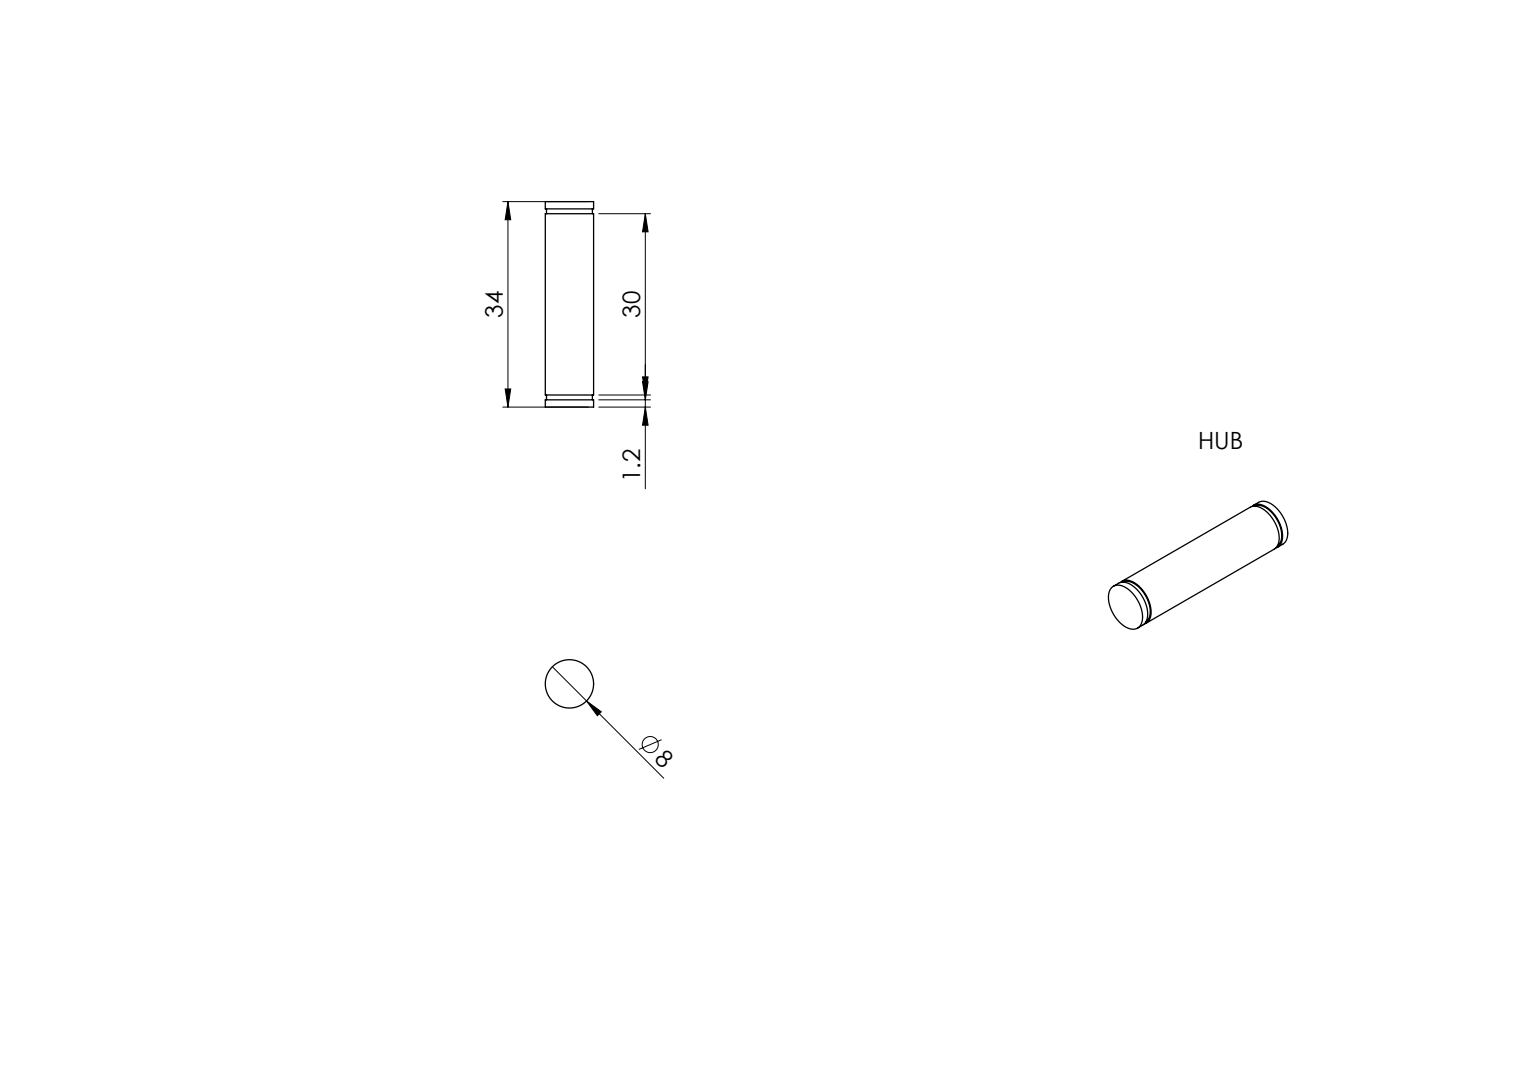
ISO-10303-21;
HEADER;
FILE_DESCRIPTION (('STEP AP214'),
    '1' );
FILE_NAME ('hub.step',
    '2026-10-31T03:44:21',
    ( '' ),
    ( '' ),
    'SwSTEP 2.0',
    'SolidWorks 2026',
    '' );
FILE_SCHEMA (( 'AUTOMOTIVE_DESIGN' ));
ENDSEC;

DATA;
#3=DIRECTION ( 'NONE',  ( -0.9999670257950099561, -0.008120795692649453515, 0.000000000000000000 ) ) ;
#38=VECTOR ( 'NONE', #9468, 1000.000000000000000 ) ;
#87=CARTESIAN_POINT ( 'NONE',  ( -155.0676494111543491, -18.79939778875158396, -15.79999999999999893 ) ) ;
#88=VERTEX_POINT ( 'NONE', #4235 ) ;
#158=AXIS2_PLACEMENT_3D ( 'NONE', #16967, #16677, #18346 ) ;
#163=DIRECTION ( 'NONE',  ( -0.9999670257950099561, -0.008120795692649453515, 0.000000000000000000 ) ) ;
#175=DIRECTION ( 'NONE',  ( 1.000000000000000000, 0.000000000000000000, 0.000000000000000000 ) ) ;
#223=DIRECTION ( 'NONE',  ( 2.191393683118470056E-17, 7.538405132783724027E-17, 1.000000000000000000 ) ) ;
#238=AXIS2_PLACEMENT_3D ( 'NONE', #6880, #15913, #19069 ) ;
#251=CIRCLE ( 'NONE', #8059, 3.800000000000000266 ) ;
#262=CARTESIAN_POINT ( 'NONE',  ( -154.9999999999999716, -14.99999999999999645, 15.79999999999999893 ) ) ;
#295=EDGE_CURVE ( 'NONE', #1806, #3807, #8927, .T. ) ;
#353=AXIS2_PLACEMENT_3D ( 'NONE', #12946, #2182, #2381 ) ;
#385=FACE_OUTER_BOUND ( 'NONE', #2616, .T. ) ;
#398=DIRECTION ( 'NONE',  ( 0.000000000000000000, 0.000000000000000000, 1.000000000000000000 ) ) ;
#423=EDGE_CURVE ( 'NONE', #3823, #976, #17703, .T. ) ;
#435=VECTOR ( 'NONE', #5633, 1000.000000000000000 ) ;
#465=EDGE_CURVE ( 'NONE', #17166, #14477, #13781, .T. ) ;
#471=ORIENTED_EDGE ( 'NONE', *, *, #4498, .F. ) ;
#479=DIRECTION ( 'NONE',  ( 0.9999419836444144449, 0.01077169184824096695, 0.000000000000000000 ) ) ;
#516=AXIS2_PLACEMENT_3D ( 'NONE', #18287, #3472, #2000 ) ;
#573=DIRECTION ( 'NONE',  ( -0.02045300604585054485, -0.9997908153927441699, -2.853726094247054863E-17 ) ) ;
#577=DIRECTION ( 'NONE',  ( -0.9999670257950099561, -0.008120795692649453515, 0.000000000000000000 ) ) ;
#594=DIRECTION ( 'NONE',  ( -0.000000000000000000, -0.000000000000000000, -1.000000000000000000 ) ) ;
#670=EDGE_CURVE ( 'NONE', #10950, #14856, #10929, .T. ) ;
#719=( NAMED_UNIT ( * ) SI_UNIT ( $, .STERADIAN. ) SOLID_ANGLE_UNIT ( ) );
#771=AXIS2_PLACEMENT_3D ( 'NONE', #7468, #11769, #12166 ) ;
#778=DIRECTION ( 'NONE',  ( 0.9999419836444144449, 0.01077169184824096695, 0.000000000000000000 ) ) ;
#833=ORIENTED_EDGE ( 'NONE', *, *, #15508, .T. ) ;
#856=CARTESIAN_POINT ( 'NONE',  ( -154.8505191518487152, -18.79705879280739467, -15.00000000000000000 ) ) ;
#867=CIRCLE ( 'NONE', #238, 4.000000000000021316 ) ;
#876=ADVANCED_FACE ( 'NONE', ( #9941 ), #2806, .F. ) ;
#964=VECTOR ( 'NONE', #1344, 1000.000000000000000 ) ;
#976=VERTEX_POINT ( 'NONE', #18201 ) ;
#979=AXIS2_PLACEMENT_3D ( 'NONE', #2910, #7500, #10431 ) ;
#994=VECTOR ( 'NONE', #12505, 999.9999999999998863 ) ;
#1010=EDGE_CURVE ( 'NONE', #13080, #4857, #251, .T. ) ;
#1011=EDGE_CURVE ( 'NONE', #88, #15786, #6202, .T. ) ;
#1029=VERTEX_POINT ( 'NONE', #10903 ) ;
#1037=CARTESIAN_POINT ( 'NONE',  ( -154.9999999999999716, -14.99999999999999645, 15.79999999999999893 ) ) ;
#1163=DIRECTION ( 'NONE',  ( 0.9999419836444144449, 0.01077169184824073971, -2.272467923560868285E-17 ) ) ;
#1171=CARTESIAN_POINT ( 'NONE',  ( -159.0000000000000000, -14.99999999999999645, -15.00000000000000000 ) ) ;
#1237=ORIENTED_EDGE ( 'NONE', *, *, #13531, .F. ) ;
#1253=ORIENTED_EDGE ( 'NONE', *, *, #5246, .T. ) ;
#1277=CARTESIAN_POINT ( 'NONE',  ( -155.0712099064782876, -18.99936609342274707, -15.79999999999999538 ) ) ;
#1342=DIRECTION ( 'NONE',  ( 0.000000000000000000, -1.000000000000000000, 0.000000000000000000 ) ) ;
#1344=DIRECTION ( 'NONE',  ( 2.191393683118470056E-17, 7.538405132783724027E-17, 1.000000000000000000 ) ) ;
#1377=EDGE_CURVE ( 'NONE', #14477, #19163, #867, .T. ) ;
#1399=DIRECTION ( 'NONE',  ( 0.000000000000000000, -1.000000000000000000, 0.000000000000000000 ) ) ;
#1407=VECTOR ( 'NONE', #12245, 1000.000000000000000 ) ;
#1410=DIRECTION ( 'NONE',  ( -0.000000000000000000, -0.000000000000000000, -1.000000000000000000 ) ) ;
#1437=LINE ( 'NONE', #5948, #15809 ) ;
#1480=ADVANCED_BREP_SHAPE_REPRESENTATION ( '', ( #8823, #10359 ), #8423 ) ;
#1486=EDGE_CURVE ( 'NONE', #976, #17995, #14820, .T. ) ;
#1506=FILL_AREA_STYLE_COLOUR ( '', #10923 ) ;
#1520=CIRCLE ( 'NONE', #16559, 4.000000000000031086 ) ;
#1522=DIRECTION ( 'NONE',  ( 0.000000000000000000, -1.000000000000000000, 0.000000000000000000 ) ) ;
#1534=DIRECTION ( 'NONE',  ( -0.000000000000000000, -0.000000000000000000, -1.000000000000000000 ) ) ;
#1551=CIRCLE ( 'NONE', #9363, 3.800000000000000266 ) ;
#1571=EDGE_LOOP ( 'NONE', ( #18455, #8024, #11206, #15769 ) ) ;
#1699=CARTESIAN_POINT ( 'NONE',  ( -150.9999999999999432, -14.99999999999999645, -15.79999999999999538 ) ) ;
#1740=( GEOMETRIC_REPRESENTATION_CONTEXT ( 3 ) GLOBAL_UNCERTAINTY_ASSIGNED_CONTEXT ( ( #16964 ) ) GLOBAL_UNIT_ASSIGNED_CONTEXT ( ( #13852, #6690, #719 ) ) REPRESENTATION_CONTEXT ( 'NONE', 'WORKASPACE' ) );
#1747=LINE ( 'NONE', #17038, #38 ) ;
#1750=VERTEX_POINT ( 'NONE', #7058 ) ;
#1787=AXIS2_PLACEMENT_3D ( 'NONE', #1037, #18895, #5430 ) ;
#1806=VERTEX_POINT ( 'NONE', #8533 ) ;
#1827=AXIS2_PLACEMENT_3D ( 'NONE', #10171, #6070, #13414 ) ;
#1886=CARTESIAN_POINT ( 'NONE',  ( -150.9999999999999432, -14.99999999999999645, 17.00000000000000000 ) ) ;
#1932=AXIS2_PLACEMENT_3D ( 'NONE', #7610, #4581, #163 ) ;
#1993=ORIENTED_EDGE ( 'NONE', *, *, #14194, .F. ) ;
#2000=DIRECTION ( 'NONE',  ( 0.000000000000000000, -1.000000000000000000, 0.000000000000000000 ) ) ;
#2045=CARTESIAN_POINT ( 'NONE',  ( -154.8605857259444463, -18.79744172571344762, 15.79999999999999893 ) ) ;
#2053=CARTESIAN_POINT ( 'NONE',  ( -155.0777214229742071, -18.79920509849242549, 15.79999999999999893 ) ) ;
#2182=DIRECTION ( 'NONE',  ( -0.000000000000000000, -0.000000000000000000, -1.000000000000000000 ) ) ;
#2216=CARTESIAN_POINT ( 'NONE',  ( -151.2002204621512078, -14.95906757097668027, -15.79999999999999893 ) ) ;
#2253=DIRECTION ( 'NONE',  ( 2.191393683118470056E-17, 7.538405132783724027E-17, 1.000000000000000000 ) ) ;
#2273=ORIENTED_EDGE ( 'NONE', *, *, #14413, .F. ) ;
#2381=DIRECTION ( 'NONE',  ( -1.000000000000000000, 0.000000000000000000, 0.000000000000000000 ) ) ;
#2384=EDGE_CURVE ( 'NONE', #4462, #5527, #16668, .T. ) ;
#2404=EDGE_CURVE ( 'NONE', #17995, #15708, #18515, .T. ) ;
#2411=CARTESIAN_POINT ( 'NONE',  ( -154.8426517387881347, -18.99690399242885874, -15.79999999999999538 ) ) ;
#2415=ORIENTED_EDGE ( 'NONE', *, *, #3275, .T. ) ;
#2432=DIRECTION ( 'NONE',  ( -0.9999670257950099561, -0.008120795692649453515, 0.000000000000000000 ) ) ;
#2462=DIRECTION ( 'NONE',  ( -2.191393683118470056E-17, -7.538405132783724027E-17, -1.000000000000000000 ) ) ;
#2558=CARTESIAN_POINT ( 'NONE',  ( -154.9999999999999716, -14.99999999999999645, -15.00000000000000000 ) ) ;
#2600=CARTESIAN_POINT ( 'NONE',  ( -158.7997795378487353, -15.04093242902330907, -15.79999999999999893 ) ) ;
#2616=EDGE_LOOP ( 'NONE', ( #12882, #6834, #7414, #8836 ) ) ;
#2634=ORIENTED_EDGE ( 'NONE', *, *, #11770, .F. ) ;
#2662=DIRECTION ( 'NONE',  ( -0.03668796685672145313, 0.9993267699245927949, 2.695122805014889898E-17 ) ) ;
#2731=LINE ( 'NONE', #2918, #7805 ) ;
#2736=ORIENTED_EDGE ( 'NONE', *, *, #4601, .T. ) ;
#2746=DIRECTION ( 'NONE',  ( 0.000000000000000000, 0.000000000000000000, -1.000000000000000000 ) ) ;
#2758=ORIENTED_EDGE ( 'NONE', *, *, #1011, .F. ) ;
#2760=CARTESIAN_POINT ( 'NONE',  ( -154.8532481325730998, -18.99730707969839116, 15.79999999999999893 ) ) ;
#2774=EDGE_LOOP ( 'NONE', ( #1993, #2634, #2415, #14369 ) ) ;
#2781=CARTESIAN_POINT ( 'NONE',  ( -154.9999999999999716, -14.99999999999999645, -15.79999999999999538 ) ) ;
#2806=PLANE ( 'NONE',  #12919 ) ;
#2868=CARTESIAN_POINT ( 'NONE',  ( -150.9999999999999432, -14.99999999999999645, 15.00000000000000000 ) ) ;
#2870=CARTESIAN_POINT ( 'NONE',  ( -151.2001253019789431, -14.96914097636792818, 15.00000000000000000 ) ) ;
#2871=CARTESIAN_POINT ( 'NONE',  ( 0.000000000000000000, 0.000000000000000000, 0.000000000000000000 ) ) ;
#2888=APPLICATION_CONTEXT ( 'automotive_design' ) ;
#2910=CARTESIAN_POINT ( 'NONE',  ( -154.9999999999999716, -14.99999999999999645, 15.79999999999999893 ) ) ;
#2911=FACE_OUTER_BOUND ( 'NONE', #4695, .T. ) ;
#2918=CARTESIAN_POINT ( 'NONE',  ( -154.8605857259444463, -18.79744172571344762, 15.00000000000000000 ) ) ;
#2983=SURFACE_STYLE_USAGE ( .BOTH. , #10055 ) ;
#2986=MECHANICAL_DESIGN_GEOMETRIC_PRESENTATION_REPRESENTATION('',(#8613),#1740);
#3058=VECTOR ( 'NONE', #18196, 1000.000000000000000 ) ;
#3081=EDGE_CURVE ( 'NONE', #3823, #4857, #6620, .T. ) ;
#3086=FILL_AREA_STYLE ('',( #1506 ) ) ;
#3190=CARTESIAN_POINT ( 'NONE',  ( -154.8505191518487152, -18.79705879280739467, -15.79999999999999893 ) ) ;
#3220=CARTESIAN_POINT ( 'NONE',  ( -154.8505191518487152, -18.79705879280739467, -15.79999999999999893 ) ) ;
#3244=EDGE_CURVE ( 'NONE', #16758, #5231, #4518, .T. ) ;
#3275=EDGE_CURVE ( 'NONE', #3719, #8297, #11699, .T. ) ;
#3295=AXIS2_PLACEMENT_3D ( 'NONE', #16109, #6193, #5104 ) ;
#3303=ORIENTED_EDGE ( 'NONE', *, *, #295, .T. ) ;
#3313=CARTESIAN_POINT ( 'NONE',  ( -155.0777214229742071, -18.79920509849242549, 15.00000000000000000 ) ) ;
#3436=ORIENTED_EDGE ( 'NONE', *, *, #423, .F. ) ;
#3438=DIRECTION ( 'NONE',  ( 1.000000000000000000, 0.000000000000000000, 0.000000000000000000 ) ) ;
#3472=DIRECTION ( 'NONE',  ( 2.191393683118470056E-17, 7.538405132783724027E-17, 1.000000000000000000 ) ) ;
#3521=PLANE ( 'NONE',  #3915 ) ;
#3588=AXIS2_PLACEMENT_3D ( 'NONE', #2781, #4732, #1399 ) ;
#3592=CARTESIAN_POINT ( 'NONE',  ( -159.0000000000000000, -14.99999999999999645, 17.00000000000000000 ) ) ;
#3686=CARTESIAN_POINT ( 'NONE',  ( -154.8505191518487152, -18.79705879280739467, -15.79999999999999893 ) ) ;
#3719=VERTEX_POINT ( 'NONE', #8643 ) ;
#3744=ORIENTED_EDGE ( 'NONE', *, *, #6811, .F. ) ;
#3750=EDGE_CURVE ( 'NONE', #976, #4855, #11582, .T. ) ;
#3807=VERTEX_POINT ( 'NONE', #2600 ) ;
#3808=CARTESIAN_POINT ( 'NONE',  ( -151.2002204621512078, -14.95906757097668027, -15.79999999999999893 ) ) ;
#3810=DIRECTION ( 'NONE',  ( -0.000000000000000000, -0.000000000000000000, -1.000000000000000000 ) ) ;
#3823=VERTEX_POINT ( 'NONE', #8843 ) ;
#3832=EDGE_CURVE ( 'NONE', #8753, #9638, #14850, .T. ) ;
#3869=FACE_OUTER_BOUND ( 'NONE', #4573, .T. ) ;
#3876=LINE ( 'NONE', #11406, #16818 ) ;
#3879=DIRECTION ( 'NONE',  ( 0.000000000000000000, 0.000000000000000000, 1.000000000000000000 ) ) ;
#3880=ADVANCED_FACE ( 'NONE', ( #10496 ), #7375, .T. ) ;
#3883=DIRECTION ( 'NONE',  ( 0.000000000000000000, 0.000000000000000000, 1.000000000000000000 ) ) ;
#3915=AXIS2_PLACEMENT_3D ( 'NONE', #2053, #8016, #573 ) ;
#3929=CARTESIAN_POINT ( 'NONE',  ( -154.9999999999999716, -14.99999999999999645, -15.79999999999999538 ) ) ;
#3933=VECTOR ( 'NONE', #18263, 1000.000000000000114 ) ;
#3949=DIRECTION ( 'NONE',  ( 2.191393683118470056E-17, 7.538405132783724027E-17, 1.000000000000000000 ) ) ;
#3981=CIRCLE ( 'NONE', #1787, 3.800000000000000266 ) ;
#3988=CARTESIAN_POINT ( 'NONE',  ( -159.0000000000000000, -14.99999999999999645, 15.79999999999999893 ) ) ;
#4008=EDGE_CURVE ( 'NONE', #7334, #15786, #12450, .T. ) ;
#4025=DIRECTION ( 'NONE',  ( 2.191393683118470056E-17, 7.538405132783724027E-17, 1.000000000000000000 ) ) ;
#4046=CARTESIAN_POINT ( 'NONE',  ( -154.9999999999999716, -14.99999999999999645, -15.79999999999999893 ) ) ;
#4054=CARTESIAN_POINT ( 'NONE',  ( -154.8532481325730998, -18.99730707969838761, 17.00000000000000000 ) ) ;
#4235=CARTESIAN_POINT ( 'NONE',  ( -154.8426517387881347, -18.99690399242885874, -15.00000000000000000 ) ) ;
#4279=CARTESIAN_POINT ( 'NONE',  ( -154.9999999999999716, -14.99999999999999645, 15.00000000000000000 ) ) ;
#4282=LINE ( 'NONE', #14762, #964 ) ;
#4355=ORIENTED_EDGE ( 'NONE', *, *, #14909, .T. ) ;
#4372=ORIENTED_EDGE ( 'NONE', *, *, #3275, .F. ) ;
#4380=DIRECTION ( 'NONE',  ( -0.9999670257950099561, -0.008120795692649453515, 0.000000000000000000 ) ) ;
#4395=LINE ( 'NONE', #10361, #10447 ) ;
#4462=VERTEX_POINT ( 'NONE', #10477 ) ;
#4466=CARTESIAN_POINT ( 'NONE',  ( -154.9999999999999716, -14.99999999999999645, 15.00000000000000000 ) ) ;
#4471=CARTESIAN_POINT ( 'NONE',  ( -154.9999999999999716, -14.99999999999999645, 15.79999999999999893 ) ) ;
#4494=DIRECTION ( 'NONE',  ( 0.000000000000000000, 0.000000000000000000, 1.000000000000000000 ) ) ;
#4498=EDGE_CURVE ( 'NONE', #6955, #1750, #18651, .T. ) ;
#4518=CIRCLE ( 'NONE', #13881, 4.000000000000031086 ) ;
#4531=LINE ( 'NONE', #7461, #3933 ) ;
#4546=AXIS2_PLACEMENT_3D ( 'NONE', #13714, #11052, #479 ) ;
#4552=ORIENTED_EDGE ( 'NONE', *, *, #4590, .F. ) ;
#4569=ORIENTED_EDGE ( 'NONE', *, *, #1377, .F. ) ;
#4571=ORIENTED_EDGE ( 'NONE', *, *, #8039, .F. ) ;
#4573=EDGE_LOOP ( 'NONE', ( #14130, #9789 ) ) ;
#4581=DIRECTION ( 'NONE',  ( 0.000000000000000000, 0.000000000000000000, -1.000000000000000000 ) ) ;
#4590=EDGE_CURVE ( 'NONE', #3807, #15831, #18329, .T. ) ;
#4598=FACE_OUTER_BOUND ( 'NONE', #13539, .T. ) ;
#4601=EDGE_CURVE ( 'NONE', #5231, #13890, #4896, .T. ) ;
#4607=UNCERTAINTY_MEASURE_WITH_UNIT (LENGTH_MEASURE( 1.000000000000000082E-05 ), #13095, 'distance_accuracy_value', 'NONE');
#4614=ADVANCED_FACE ( 'NONE', ( #9294 ), #3521, .F. ) ;
#4677=VERTEX_POINT ( 'NONE', #13017 ) ;
#4695=EDGE_LOOP ( 'NONE', ( #17550, #19003, #11844, #17218, #8897, #6661, #8715, #12787 ) ) ;
#4716=AXIS2_PLACEMENT_3D ( 'NONE', #2558, #15677, #1163 ) ;
#4732=DIRECTION ( 'NONE',  ( 2.191393683118470056E-17, 7.538405132783724027E-17, 1.000000000000000000 ) ) ;
#4735=DIRECTION ( 'NONE',  ( 0.000000000000000000, 0.000000000000000000, -1.000000000000000000 ) ) ;
#4738=CARTESIAN_POINT ( 'NONE',  ( -159.0000000000000000, -14.99999999999999645, -17.00000000000000000 ) ) ;
#4832=ORIENTED_EDGE ( 'NONE', *, *, #15508, .F. ) ;
#4854=ORIENTED_EDGE ( 'NONE', *, *, #11794, .F. ) ;
#4855=VERTEX_POINT ( 'NONE', #7234 ) ;
#4857=VERTEX_POINT ( 'NONE', #5964 ) ;
#4868=EDGE_LOOP ( 'NONE', ( #12573, #13501, #16712, #6610 ) ) ;
#4896=LINE ( 'NONE', #12144, #1407 ) ;
#4940=ORIENTED_EDGE ( 'NONE', *, *, #9990, .F. ) ;
#4980=AXIS2_PLACEMENT_3D ( 'NONE', #11597, #1410, #8567 ) ;
#5001=EDGE_CURVE ( 'NONE', #8753, #5527, #4395, .T. ) ;
#5013=DIRECTION ( 'NONE',  ( -1.000000000000000000, 0.000000000000000000, 0.000000000000000000 ) ) ;
#5040=DIRECTION ( 'NONE',  ( -0.9999670257950100671, -0.008120795692649436168, -2.775557561562891043E-17 ) ) ;
#5058=FACE_OUTER_BOUND ( 'NONE', #6710, .T. ) ;
#5097=ORIENTED_EDGE ( 'NONE', *, *, #17583, .F. ) ;
#5102=PRODUCT_DEFINITION_FORMATION_WITH_SPECIFIED_SOURCE ( 'ANY', '', #7416, .NOT_KNOWN. ) ;
#5104=DIRECTION ( 'NONE',  ( 0.9999419836444144449, 0.01077169184824096695, 0.000000000000000000 ) ) ;
#5115=CARTESIAN_POINT ( 'NONE',  ( -154.9999999999999716, -14.99999999999999645, 15.79999999999999893 ) ) ;
#5164=DIRECTION ( 'NONE',  ( -0.000000000000000000, -0.000000000000000000, -1.000000000000000000 ) ) ;
#5209=EDGE_CURVE ( 'NONE', #4677, #17411, #6885, .T. ) ;
#5231=VERTEX_POINT ( 'NONE', #18875 ) ;
#5246=EDGE_CURVE ( 'NONE', #1750, #10122, #18934, .T. ) ;
#5255=AXIS2_PLACEMENT_3D ( 'NONE', #14942, #15045, #1522 ) ;
#5430=DIRECTION ( 'NONE',  ( -0.9999670257950099561, -0.008120795692649453515, 0.000000000000000000 ) ) ;
#5441=VECTOR ( 'NONE', #10017, 1000.000000000000000 ) ;
#5471=DIRECTION ( 'NONE',  ( 0.03933706530295848214, -0.9992259981072103558, 7.446367396525006349E-17 ) ) ;
#5527=VERTEX_POINT ( 'NONE', #4738 ) ;
#5533=CARTESIAN_POINT ( 'NONE',  ( -154.9999999999999716, -14.99999999999999645, -17.00000000000000000 ) ) ;
#5543=SURFACE_STYLE_FILL_AREA ( #3086 ) ;
#5633=DIRECTION ( 'NONE',  ( 0.000000000000000000, 0.000000000000000000, -1.000000000000000000 ) ) ;
#5673=ORIENTED_EDGE ( 'NONE', *, *, #17437, .T. ) ;
#5795=VECTOR ( 'NONE', #16551, 1000.000000000000000 ) ;
#5866=CLOSED_SHELL ( 'NONE', ( #19264, #12279, #18324, #11424, #7297, #14652, #9924, #9749, #15801, #876, #9900, #4614, #18642, #11325, #6067, #8324, #8547, #15027, #6184, #3880 ) ) ;
#5876=AXIS2_PLACEMENT_3D ( 'NONE', #3686, #9651, #15646 ) ;
#5948=CARTESIAN_POINT ( 'NONE',  ( -155.0818120241833640, -18.99916326157099178, 17.00000000000000000 ) ) ;
#5964=CARTESIAN_POINT ( 'NONE',  ( -158.7998746980210001, -15.03085902363206472, 15.00000000000000000 ) ) ;
#5978=EDGE_LOOP ( 'NONE', ( #14095, #13335, #8853, #6829 ) ) ;
#5980=VECTOR ( 'NONE', #13355, 1000.000000000000000 ) ;
#6006=ORIENTED_EDGE ( 'NONE', *, *, #6879, .F. ) ;
#6048=ORIENTED_EDGE ( 'NONE', *, *, #6384, .F. ) ;
#6067=ADVANCED_FACE ( 'NONE', ( #13812 ), #18349, .T. ) ;
#6070=DIRECTION ( 'NONE',  ( 0.000000000000000000, 0.000000000000000000, -1.000000000000000000 ) ) ;
#6075=FACE_OUTER_BOUND ( 'NONE', #8734, .T. ) ;
#6108=FACE_OUTER_BOUND ( 'NONE', #13171, .T. ) ;
#6184=ADVANCED_FACE ( 'NONE', ( #7140 ), #15777, .F. ) ;
#6193=DIRECTION ( 'NONE',  ( -2.191393683118470056E-17, -7.538405132783724027E-17, -1.000000000000000000 ) ) ;
#6202=CIRCLE ( 'NONE', #5255, 4.000000000000021316 ) ;
#6260=ORIENTED_EDGE ( 'NONE', *, *, #6626, .F. ) ;
#6286=APPLICATION_CONTEXT ( 'automotive_design' ) ;
#6384=EDGE_CURVE ( 'NONE', #9638, #1806, #10167, .T. ) ;
#6389=EDGE_CURVE ( 'NONE', #15708, #10950, #7208, .T. ) ;
#6455=ORIENTED_EDGE ( 'NONE', *, *, #13363, .F. ) ;
#6463=CARTESIAN_POINT ( 'NONE',  ( -150.9999999999999432, -14.99999999999999645, 15.79999999999999893 ) ) ;
#6598=AXIS2_PLACEMENT_3D ( 'NONE', #7634, #11951, #3 ) ;
#6609=CARTESIAN_POINT ( 'NONE',  ( -150.9999999999999432, -14.99999999999999645, -15.00000000000000000 ) ) ;
#6610=ORIENTED_EDGE ( 'NONE', *, *, #8951, .F. ) ;
#6620=LINE ( 'NONE', #14156, #10755 ) ;
#6626=EDGE_CURVE ( 'NONE', #3807, #6955, #1747, .T. ) ;
#6640=DIRECTION ( 'NONE',  ( -0.9993267699245929059, -0.03668796685672145313, -2.853726094247056096E-17 ) ) ;
#6661=ORIENTED_EDGE ( 'NONE', *, *, #6879, .T. ) ;
#6690=( NAMED_UNIT ( * ) PLANE_ANGLE_UNIT ( ) SI_UNIT ( $, .RADIAN. ) );
#6710=EDGE_LOOP ( 'NONE', ( #9354, #8522, #17657, #4854 ) ) ;
#6786=DIRECTION ( 'NONE',  ( -0.02045300604585054485, -0.9997908153927442809, -2.853726094247055479E-17 ) ) ;
#6811=EDGE_CURVE ( 'NONE', #7334, #4677, #15698, .T. ) ;
#6829=ORIENTED_EDGE ( 'NONE', *, *, #670, .F. ) ;
#6834=ORIENTED_EDGE ( 'NONE', *, *, #19015, .T. ) ;
#6836=DIRECTION ( 'NONE',  ( 0.000000000000000000, 0.000000000000000000, -1.000000000000000000 ) ) ;
#6879=EDGE_CURVE ( 'NONE', #1029, #3823, #16009, .T. ) ;
#6880=CARTESIAN_POINT ( 'NONE',  ( -154.9999999999999716, -14.99999999999999645, -15.79999999999999538 ) ) ;
#6885=LINE ( 'NONE', #4054, #5441 ) ;
#6924=( NAMED_UNIT ( * ) SI_UNIT ( $, .STERADIAN. ) SOLID_ANGLE_UNIT ( ) );
#6955=VERTEX_POINT ( 'NONE', #8678 ) ;
#7010=AXIS2_PLACEMENT_3D ( 'NONE', #8647, #14438, #14724 ) ;
#7052=DIRECTION ( 'NONE',  ( 0.000000000000000000, -1.000000000000000000, 0.000000000000000000 ) ) ;
#7058=CARTESIAN_POINT ( 'NONE',  ( -151.2002204621512078, -14.95906757097668027, -15.00000000000000000 ) ) ;
#7096=ORIENTED_EDGE ( 'NONE', *, *, #1486, .F. ) ;
#7118=ORIENTED_EDGE ( 'NONE', *, *, #1011, .T. ) ;
#7140=FACE_OUTER_BOUND ( 'NONE', #11044, .T. ) ;
#7208=CIRCLE ( 'NONE', #18191, 4.000000000000031086 ) ;
#7234=CARTESIAN_POINT ( 'NONE',  ( -155.0818120241833640, -18.99916326157099533, 15.79999999999999893 ) ) ;
#7297=ADVANCED_FACE ( 'NONE', ( #14416 ), #15706, .T. ) ;
#7327=DIRECTION ( 'NONE',  ( 0.9998415233556813275, -0.01780247661957949992, -2.056844117275891959E-17 ) ) ;
#7334=VERTEX_POINT ( 'NONE', #2868 ) ;
#7375=CYLINDRICAL_SURFACE ( 'NONE', #771, 3.799999999999993605 ) ;
#7414=ORIENTED_EDGE ( 'NONE', *, *, #2384, .T. ) ;
#7416=PRODUCT ( 'hub', 'hub', '', ( #8926 ) ) ;
#7461=CARTESIAN_POINT ( 'NONE',  ( -155.0676494111543491, -18.79939778875158396, -15.00000000000000000 ) ) ;
#7468=CARTESIAN_POINT ( 'NONE',  ( -154.9999999999999716, -14.99999999999999645, -15.79999999999999893 ) ) ;
#7500=DIRECTION ( 'NONE',  ( 0.000000000000000000, 0.000000000000000000, 1.000000000000000000 ) ) ;
#7545=CIRCLE ( 'NONE', #9410, 4.000000000000021316 ) ;
#7610=CARTESIAN_POINT ( 'NONE',  ( -154.9999999999999716, -14.99999999999999645, 15.79999999999999893 ) ) ;
#7634=CARTESIAN_POINT ( 'NONE',  ( -154.9999999999999716, -14.99999999999999645, 15.00000000000000000 ) ) ;
#7653=EDGE_CURVE ( 'NONE', #15786, #14856, #14923, .T. ) ;
#7671=CIRCLE ( 'NONE', #11726, 4.000000000000021316 ) ;
#7805=VECTOR ( 'NONE', #11914, 1000.000000000000114 ) ;
#7837=AXIS2_PLACEMENT_3D ( 'NONE', #18634, #9298, #577 ) ;
#7864=CARTESIAN_POINT ( 'NONE',  ( -154.9999999999999716, -14.99999999999999645, -15.79999999999999893 ) ) ;
#7983=ORIENTED_EDGE ( 'NONE', *, *, #2384, .F. ) ;
#8009=ORIENTED_EDGE ( 'NONE', *, *, #5246, .F. ) ;
#8010=CARTESIAN_POINT ( 'NONE',  ( -150.9999999999999432, -14.99999999999999645, 17.00000000000000000 ) ) ;
#8014=CARTESIAN_POINT ( 'NONE',  ( -154.9999999999999716, -14.99999999999999645, 15.79999999999999893 ) ) ;
#8016=DIRECTION ( 'NONE',  ( 0.9997908153927442809, -0.02045300604585054832, 2.695122805014890206E-17 ) ) ;
#8024=ORIENTED_EDGE ( 'NONE', *, *, #11061, .T. ) ;
#8037=AXIS2_PLACEMENT_3D ( 'NONE', #8014, #6836, #11243 ) ;
#8039=EDGE_CURVE ( 'NONE', #9546, #17411, #14616, .T. ) ;
#8059=AXIS2_PLACEMENT_3D ( 'NONE', #4466, #13477, #8959 ) ;
#8071=ORIENTED_EDGE ( 'NONE', *, *, #9921, .F. ) ;
#8115=( GEOMETRIC_REPRESENTATION_CONTEXT ( 3 ) GLOBAL_UNCERTAINTY_ASSIGNED_CONTEXT ( ( #4607 ) ) GLOBAL_UNIT_ASSIGNED_CONTEXT ( ( #13095, #19107, #13462 ) ) REPRESENTATION_CONTEXT ( 'NONE', 'WORKASPACE' ) );
#8270=ORIENTED_EDGE ( 'NONE', *, *, #1010, .F. ) ;
#8286=ORIENTED_EDGE ( 'NONE', *, *, #1010, .T. ) ;
#8288=ORIENTED_EDGE ( 'NONE', *, *, #3081, .T. ) ;
#8297=VERTEX_POINT ( 'NONE', #13402 ) ;
#8324=ADVANCED_FACE ( 'NONE', ( #16259 ), #8798, .F. ) ;
#8340=DIRECTION ( 'NONE',  ( -1.000000000000000000, 0.000000000000000000, 0.000000000000000000 ) ) ;
#8423=( GEOMETRIC_REPRESENTATION_CONTEXT ( 3 ) GLOBAL_UNCERTAINTY_ASSIGNED_CONTEXT ( ( #16383 ) ) GLOBAL_UNIT_ASSIGNED_CONTEXT ( ( #13001, #19007, #6924 ) ) REPRESENTATION_CONTEXT ( 'NONE', 'WORKASPACE' ) );
#8493=CYLINDRICAL_SURFACE ( 'NONE', #8750, 3.800000000000000266 ) ;
#8522=ORIENTED_EDGE ( 'NONE', *, *, #11972, .T. ) ;
#8533=CARTESIAN_POINT ( 'NONE',  ( -155.0676494111543491, -18.79939778875158396, -15.79999999999999893 ) ) ;
#8547=ADVANCED_FACE ( 'NONE', ( #5058 ), #14159, .F. ) ;
#8567=DIRECTION ( 'NONE',  ( -1.000000000000000000, 0.000000000000000000, 0.000000000000000000 ) ) ;
#8574=DIRECTION ( 'NONE',  ( 0.000000000000000000, 0.000000000000000000, 1.000000000000000000 ) ) ;
#8590=ORIENTED_EDGE ( 'NONE', *, *, #10467, .F. ) ;
#8613=STYLED_ITEM('',(#19482),#8823);
#8643=CARTESIAN_POINT ( 'NONE',  ( -154.8605857259444463, -18.79744172571344762, 15.79999999999999893 ) ) ;
#8647=CARTESIAN_POINT ( 'NONE',  ( -154.9999999999999716, -14.99999999999999645, -15.00000000000000000 ) ) ;
#8678=CARTESIAN_POINT ( 'NONE',  ( -158.7997795378487353, -15.04093242902330907, -15.00000000000000000 ) ) ;
#8704=AXIS2_PLACEMENT_3D ( 'NONE', #10791, #9322, #5013 ) ;
#8706=VERTEX_POINT ( 'NONE', #16333 ) ;
#8715=ORIENTED_EDGE ( 'NONE', *, *, #423, .T. ) ;
#8717=CIRCLE ( 'NONE', #1827, 4.000000000000031086 ) ;
#8719=PRODUCT_DEFINITION_CONTEXT ( 'detailed design', #6286, 'design' ) ;
#8734=EDGE_LOOP ( 'NONE', ( #17536, #18258, #2736, #15788, #14951, #19210, #8898, #14886, #12932, #18010, #15244, #19234, #12730, #4569, #9076, #7118, #15263, #18210, #19137, #4571 ) ) ;
#8750=AXIS2_PLACEMENT_3D ( 'NONE', #15846, #17523, #2432 ) ;
#8753=VERTEX_POINT ( 'NONE', #15137 ) ;
#8761=AXIS2_PLACEMENT_3D ( 'NONE', #4471, #15432, #5040 ) ;
#8767=DIRECTION ( 'NONE',  ( 1.000000000000000000, 0.000000000000000000, -0.000000000000000000 ) ) ;
#8798=PLANE ( 'NONE',  #13380 ) ;
#8823=MANIFOLD_SOLID_BREP ( 'Cavity1', #5866 ) ;
#8834=DIRECTION ( 'NONE',  ( 0.000000000000000000, 0.000000000000000000, 1.000000000000000000 ) ) ;
#8836=ORIENTED_EDGE ( 'NONE', *, *, #5001, .F. ) ;
#8843=CARTESIAN_POINT ( 'NONE',  ( -158.7998746980210001, -15.03085902363206472, 15.79999999999999893 ) ) ;
#8853=ORIENTED_EDGE ( 'NONE', *, *, #7653, .T. ) ;
#8872=PLANE ( 'NONE',  #8761 ) ;
#8878=CARTESIAN_POINT ( 'NONE',  ( -154.9999999999999716, -14.99999999999999645, -15.00000000000000000 ) ) ;
#8884=DIRECTION ( 'NONE',  ( 2.775466039758894710E-17, 2.253973589064049552E-19, -1.000000000000000000 ) ) ;
#8897=ORIENTED_EDGE ( 'NONE', *, *, #11770, .T. ) ;
#8898=ORIENTED_EDGE ( 'NONE', *, *, #670, .T. ) ;
#8926=PRODUCT_CONTEXT ( 'NONE', #2888, 'mechanical' ) ;
#8927=CIRCLE ( 'NONE', #3295, 3.799999999999993605 ) ;
#8928=EDGE_CURVE ( 'NONE', #14856, #8706, #7671, .T. ) ;
#8951=EDGE_CURVE ( 'NONE', #4855, #15708, #1437, .T. ) ;
#8959=DIRECTION ( 'NONE',  ( -0.9999670257950099561, -0.008120795692649453515, 0.000000000000000000 ) ) ;
#8998=PLANE ( 'NONE',  #12789 ) ;
#9076=ORIENTED_EDGE ( 'NONE', *, *, #11794, .T. ) ;
#9178=DIRECTION ( 'NONE',  ( -0.9999670257950100671, -0.008120795692649436168, -2.775557561562891043E-17 ) ) ;
#9283=EDGE_CURVE ( 'NONE', #8706, #12622, #4531, .T. ) ;
#9294=FACE_OUTER_BOUND ( 'NONE', #4868, .T. ) ;
#9298=DIRECTION ( 'NONE',  ( 0.000000000000000000, 0.000000000000000000, -1.000000000000000000 ) ) ;
#9300=AXIS2_PLACEMENT_3D ( 'NONE', #4046, #3949, #15908 ) ;
#9322=DIRECTION ( 'NONE',  ( 0.000000000000000000, 0.000000000000000000, -1.000000000000000000 ) ) ;
#9333=ORIENTED_EDGE ( 'NONE', *, *, #465, .T. ) ;
#9354=ORIENTED_EDGE ( 'NONE', *, *, #465, .F. ) ;
#9363=AXIS2_PLACEMENT_3D ( 'NONE', #4279, #13198, #4380 ) ;
#9410=AXIS2_PLACEMENT_3D ( 'NONE', #3929, #4025, #7052 ) ;
#9468=DIRECTION ( 'NONE',  ( 2.191393683118470056E-17, 7.538405132783724027E-17, 1.000000000000000000 ) ) ;
#9546=VERTEX_POINT ( 'NONE', #6463 ) ;
#9564=AXIS2_PLACEMENT_3D ( 'NONE', #12419, #5164, #14079 ) ;
#9570=CARTESIAN_POINT ( 'NONE',  ( -155.0712099064782876, -18.99936609342274352, 17.00000000000000000 ) ) ;
#9638=VERTEX_POINT ( 'NONE', #1277 ) ;
#9651=DIRECTION ( 'NONE',  ( -0.9992259981072103558, -0.03933706530295846826, 2.486236275248362725E-17 ) ) ;
#9726=PRODUCT_DEFINITION ( 'UNKNOWN', '', #5102, #8719 ) ;
#9748=DIRECTION ( 'NONE',  ( 0.000000000000000000, 0.000000000000000000, -1.000000000000000000 ) ) ;
#9749=ADVANCED_FACE ( 'NONE', ( #6075 ), #12236, .T. ) ;
#9764=ORIENTED_EDGE ( 'NONE', *, *, #14194, .T. ) ;
#9788=DIRECTION ( 'NONE',  ( -2.191393683118470056E-17, -7.538405132783724027E-17, -1.000000000000000000 ) ) ;
#9789=ORIENTED_EDGE ( 'NONE', *, *, #3244, .T. ) ;
#9813=ORIENTED_EDGE ( 'NONE', *, *, #14844, .F. ) ;
#9829=DIRECTION ( 'NONE',  ( 0.000000000000000000, 0.000000000000000000, 1.000000000000000000 ) ) ;
#9877=LINE ( 'NONE', #11447, #18134 ) ;
#9900=ADVANCED_FACE ( 'NONE', ( #17242 ), #15563, .F. ) ;
#9921=EDGE_CURVE ( 'NONE', #15831, #1750, #12617, .T. ) ;
#9924=ADVANCED_FACE ( 'NONE', ( #385 ), #18624, .T. ) ;
#9941=FACE_OUTER_BOUND ( 'NONE', #11396, .T. ) ;
#9990=EDGE_CURVE ( 'NONE', #8706, #9638, #18718, .T. ) ;
#10017=DIRECTION ( 'NONE',  ( 0.000000000000000000, 0.000000000000000000, 1.000000000000000000 ) ) ;
#10030=CARTESIAN_POINT ( 'NONE',  ( -154.9999999999999716, -14.99999999999999645, 17.00000000000000000 ) ) ;
#10055=SURFACE_SIDE_STYLE ('',( #5543 ) ) ;
#10064=AXIS2_PLACEMENT_3D ( 'NONE', #10934, #15259, #175 ) ;
#10103=SHAPE_DEFINITION_REPRESENTATION ( #13356, #14681 ) ;
#10122=VERTEX_POINT ( 'NONE', #856 ) ;
#10148=ORIENTED_EDGE ( 'NONE', *, *, #12522, .T. ) ;
#10167=LINE ( 'NONE', #87, #15051 ) ;
#10171=CARTESIAN_POINT ( 'NONE',  ( -154.9999999999999716, -14.99999999999999645, 15.00000000000000000 ) ) ;
#10227=DIRECTION ( 'NONE',  ( 1.000000000000000000, 0.000000000000000000, 0.000000000000000000 ) ) ;
#10359=AXIS2_PLACEMENT_3D ( 'NONE', #2871, #8834, #16191 ) ;
#10361=CARTESIAN_POINT ( 'NONE',  ( -159.0000000000000000, -14.99999999999999645, 17.00000000000000000 ) ) ;
#10407=VECTOR ( 'NONE', #16935, 1000.000000000000000 ) ;
#10431=DIRECTION ( 'NONE',  ( -0.9999670257950099561, -0.008120795692649453515, 0.000000000000000000 ) ) ;
#10447=VECTOR ( 'NONE', #13509, 1000.000000000000000 ) ;
#10467=EDGE_CURVE ( 'NONE', #1806, #12622, #4282, .T. ) ;
#10477=CARTESIAN_POINT ( 'NONE',  ( -150.9999999999999432, -14.99999999999999645, -17.00000000000000000 ) ) ;
#10489=AXIS2_PLACEMENT_3D ( 'NONE', #262, #4494, #14968 ) ;
#10496=FACE_OUTER_BOUND ( 'NONE', #11593, .T. ) ;
#10538=PLANE ( 'NONE',  #11937 ) ;
#10656=EDGE_LOOP ( 'NONE', ( #833, #4372, #9813, #14583 ) ) ;
#10755=VECTOR ( 'NONE', #9748, 1000.000000000000000 ) ;
#10791=CARTESIAN_POINT ( 'NONE',  ( -154.9999999999999716, -14.99999999999999645, 15.79999999999999893 ) ) ;
#10829=ORIENTED_EDGE ( 'NONE', *, *, #295, .F. ) ;
#10843=ORIENTED_EDGE ( 'NONE', *, *, #1377, .T. ) ;
#10849=DIRECTION ( 'NONE',  ( -0.000000000000000000, -0.000000000000000000, -1.000000000000000000 ) ) ;
#10891=SHAPE_REPRESENTATION_RELATIONSHIP ( 'NONE' , 'NONE' ,  #14681, #1480 ) ;
#10903=CARTESIAN_POINT ( 'NONE',  ( -151.2001253019789431, -14.96914097636792818, 15.79999999999999893 ) ) ;
#10923=COLOUR_RGB ( '',0.8941176470588234615, 0.8941176470588234615, 0.8941176470588234615 ) ;
#10929=LINE ( 'NONE', #3592, #10407 ) ;
#10932=CIRCLE ( 'NONE', #15337, 4.000000000000031086 ) ;
#10934=CARTESIAN_POINT ( 'NONE',  ( -154.9999999999999716, -14.99999999999999645, -17.00000000000000000 ) ) ;
#10950=VERTEX_POINT ( 'NONE', #11990 ) ;
#11044=EDGE_LOOP ( 'NONE', ( #6455, #8009, #471, #15505, #14688, #18870, #13860, #2758 ) ) ;
#11052=DIRECTION ( 'NONE',  ( -2.191393683118470056E-17, -7.538405132783724027E-17, -1.000000000000000000 ) ) ;
#11061=EDGE_CURVE ( 'NONE', #16758, #9546, #17052, .T. ) ;
#11185=CYLINDRICAL_SURFACE ( 'NONE', #9300, 3.799999999999993605 ) ;
#11206=ORIENTED_EDGE ( 'NONE', *, *, #12790, .F. ) ;
#11243=DIRECTION ( 'NONE',  ( -1.000000000000000000, 0.000000000000000000, 0.000000000000000000 ) ) ;
#11261=CARTESIAN_POINT ( 'NONE',  ( -154.8505191518487152, -18.79705879280739467, -15.79999999999999893 ) ) ;
#11325=ADVANCED_FACE ( 'NONE', ( #11920 ), #10538, .F. ) ;
#11396=EDGE_LOOP ( 'NONE', ( #2273, #7983 ) ) ;
#11406=CARTESIAN_POINT ( 'NONE',  ( -154.8426517387881347, -18.99690399242885874, 17.00000000000000000 ) ) ;
#11424=ADVANCED_FACE ( 'NONE', ( #12210 ), #18020, .T. ) ;
#11447=CARTESIAN_POINT ( 'NONE',  ( -154.8505191518487152, -18.79705879280739467, -15.00000000000000000 ) ) ;
#11519=PRESENTATION_STYLE_ASSIGNMENT (( #2983 ) ) ;
#11582=LINE ( 'NONE', #14520, #12032 ) ;
#11593=EDGE_LOOP ( 'NONE', ( #6260, #10829, #18046, #4355 ) ) ;
#11597=CARTESIAN_POINT ( 'NONE',  ( -154.9999999999999716, -14.99999999999999645, 17.00000000000000000 ) ) ;
#11616=CARTESIAN_POINT ( 'NONE',  ( -154.9999999999999716, -14.99999999999999645, 15.00000000000000000 ) ) ;
#11699=LINE ( 'NONE', #15938, #435 ) ;
#11726=AXIS2_PLACEMENT_3D ( 'NONE', #8878, #13290, #1342 ) ;
#11769=DIRECTION ( 'NONE',  ( 2.191393683118470056E-17, 7.538405132783724027E-17, 1.000000000000000000 ) ) ;
#11770=EDGE_CURVE ( 'NONE', #3719, #1029, #3981, .T. ) ;
#11794=EDGE_CURVE ( 'NONE', #14477, #88, #3876, .T. ) ;
#11844=ORIENTED_EDGE ( 'NONE', *, *, #8039, .T. ) ;
#11914=DIRECTION ( 'NONE',  ( -0.03668796685672145313, 0.9993267699245927949, 2.695122805014889898E-17 ) ) ;
#11920=FACE_OUTER_BOUND ( 'NONE', #12320, .T. ) ;
#11937=AXIS2_PLACEMENT_3D ( 'NONE', #19315, #8884, #9178 ) ;
#11951=DIRECTION ( 'NONE',  ( 0.000000000000000000, 0.000000000000000000, 1.000000000000000000 ) ) ;
#11972=EDGE_CURVE ( 'NONE', #17166, #10122, #17996, .T. ) ;
#11990=CARTESIAN_POINT ( 'NONE',  ( -159.0000000000000000, -14.99999999999999645, 15.00000000000000000 ) ) ;
#12032=VECTOR ( 'NONE', #6786, 999.9999999999998863 ) ;
#12079=DIRECTION ( 'NONE',  ( 0.9999419836444144449, 0.01077169184824096695, 0.000000000000000000 ) ) ;
#12144=CARTESIAN_POINT ( 'NONE',  ( -159.0000000000000000, -14.99999999999999645, 17.00000000000000000 ) ) ;
#12166=DIRECTION ( 'NONE',  ( 0.9999419836444144449, 0.01077169184824096695, 0.000000000000000000 ) ) ;
#12210=FACE_OUTER_BOUND ( 'NONE', #14244, .T. ) ;
#12236=CYLINDRICAL_SURFACE ( 'NONE', #14896, 4.000000000000031086 ) ;
#12245=DIRECTION ( 'NONE',  ( -0.000000000000000000, -0.000000000000000000, -1.000000000000000000 ) ) ;
#12279=ADVANCED_FACE ( 'NONE', ( #18869 ), #11185, .T. ) ;
#12320=EDGE_LOOP ( 'NONE', ( #16705, #18009, #8270, #5097, #4832, #3744, #1237, #14754 ) ) ;
#12419=CARTESIAN_POINT ( 'NONE',  ( -154.9999999999999716, -14.99999999999999645, 17.00000000000000000 ) ) ;
#12450=LINE ( 'NONE', #1886, #12662 ) ;
#12505=DIRECTION ( 'NONE',  ( -0.02045300604585054485, -0.9997908153927442809, -2.853726094247055479E-17 ) ) ;
#12522=EDGE_CURVE ( 'NONE', #15831, #17166, #18104, .T. ) ;
#12550=CIRCLE ( 'NONE', #6598, 3.800000000000000266 ) ;
#12573=ORIENTED_EDGE ( 'NONE', *, *, #3750, .F. ) ;
#12617=LINE ( 'NONE', #3808, #18052 ) ;
#12622=VERTEX_POINT ( 'NONE', #14392 ) ;
#12662=VECTOR ( 'NONE', #594, 1000.000000000000000 ) ;
#12730=ORIENTED_EDGE ( 'NONE', *, *, #19015, .F. ) ;
#12739=ORIENTED_EDGE ( 'NONE', *, *, #4498, .T. ) ;
#12787=ORIENTED_EDGE ( 'NONE', *, *, #3750, .T. ) ;
#12789=AXIS2_PLACEMENT_3D ( 'NONE', #14883, #16174, #13417 ) ;
#12790=EDGE_CURVE ( 'NONE', #13890, #9546, #15904, .T. ) ;
#12821=ORIENTED_EDGE ( 'NONE', *, *, #6626, .T. ) ;
#12882=ORIENTED_EDGE ( 'NONE', *, *, #17437, .F. ) ;
#12887=PLANE ( 'NONE',  #16276 ) ;
#12919=AXIS2_PLACEMENT_3D ( 'NONE', #5533, #3883, #8767 ) ;
#12932=ORIENTED_EDGE ( 'NONE', *, *, #9990, .T. ) ;
#12946=CARTESIAN_POINT ( 'NONE',  ( -154.9999999999999716, -14.99999999999999645, 17.00000000000000000 ) ) ;
#12978=EDGE_LOOP ( 'NONE', ( #18306, #16778, #1253, #19214 ) ) ;
#13001=( LENGTH_UNIT ( ) NAMED_UNIT ( * ) SI_UNIT ( .MILLI., .METRE. ) );
#13017=CARTESIAN_POINT ( 'NONE',  ( -154.8532481325730998, -18.99730707969839116, 15.00000000000000000 ) ) ;
#13020=AXIS2_PLACEMENT_3D ( 'NONE', #2045, #6640, #17050 ) ;
#13025=CARTESIAN_POINT ( 'NONE',  ( -154.9999999999999716, -14.99999999999999645, -15.79999999999999893 ) ) ;
#13080=VERTEX_POINT ( 'NONE', #2870 ) ;
#13095=( LENGTH_UNIT ( ) NAMED_UNIT ( * ) SI_UNIT ( .MILLI., .METRE. ) );
#13171=EDGE_LOOP ( 'NONE', ( #4552, #12821, #12739, #8071 ) ) ;
#13198=DIRECTION ( 'NONE',  ( 0.000000000000000000, 0.000000000000000000, 1.000000000000000000 ) ) ;
#13206=ORIENTED_EDGE ( 'NONE', *, *, #6384, .T. ) ;
#13241=EDGE_CURVE ( 'NONE', #5231, #16758, #1520, .T. ) ;
#13284=DIRECTION ( 'NONE',  ( 0.000000000000000000, 0.000000000000000000, -1.000000000000000000 ) ) ;
#13288=LINE ( 'NONE', #19405, #17525 ) ;
#13290=DIRECTION ( 'NONE',  ( 2.191393683118470056E-17, 7.538405132783724027E-17, 1.000000000000000000 ) ) ;
#13302=DIRECTION ( 'NONE',  ( 0.01780247661957949645, 0.9998415233556812165, -7.576222706442768103E-17 ) ) ;
#13335=ORIENTED_EDGE ( 'NONE', *, *, #4008, .T. ) ;
#13355=DIRECTION ( 'NONE',  ( -0.000000000000000000, -0.000000000000000000, -1.000000000000000000 ) ) ;
#13356=PRODUCT_DEFINITION_SHAPE ( 'NONE', 'NONE',  #9726 ) ;
#13363=EDGE_CURVE ( 'NONE', #10122, #88, #9877, .T. ) ;
#13380=AXIS2_PLACEMENT_3D ( 'NONE', #14770, #7327, #13302 ) ;
#13402=CARTESIAN_POINT ( 'NONE',  ( -154.8605857259444463, -18.79744172571344762, 15.00000000000000000 ) ) ;
#13414=DIRECTION ( 'NONE',  ( -1.000000000000000000, 0.000000000000000000, 0.000000000000000000 ) ) ;
#13417=DIRECTION ( 'NONE',  ( 0.9999419836444144449, 0.01077169184824073971, -2.272467923560868285E-17 ) ) ;
#13462=( NAMED_UNIT ( * ) SI_UNIT ( $, .STERADIAN. ) SOLID_ANGLE_UNIT ( ) );
#13477=DIRECTION ( 'NONE',  ( 0.000000000000000000, 0.000000000000000000, 1.000000000000000000 ) ) ;
#13501=ORIENTED_EDGE ( 'NONE', *, *, #1486, .T. ) ;
#13509=DIRECTION ( 'NONE',  ( -0.000000000000000000, -0.000000000000000000, -1.000000000000000000 ) ) ;
#13531=EDGE_CURVE ( 'NONE', #10950, #7334, #8717, .T. ) ;
#13539=EDGE_LOOP ( 'NONE', ( #10843, #5673, #16170, #13206, #3303, #16511, #10148, #9333 ) ) ;
#13714=CARTESIAN_POINT ( 'NONE',  ( -154.9999999999999716, -14.99999999999999645, -15.00000000000000000 ) ) ;
#13742=CYLINDRICAL_SURFACE ( 'NONE', #18195, 3.799999999999993605 ) ;
#13744=MECHANICAL_DESIGN_GEOMETRIC_PRESENTATION_REPRESENTATION('',(#18154),#8115);
#13781=LINE ( 'NONE', #3220, #5795 ) ;
#13812=FACE_OUTER_BOUND ( 'NONE', #2774, .T. ) ;
#13852=( LENGTH_UNIT ( ) NAMED_UNIT ( * ) SI_UNIT ( .MILLI., .METRE. ) );
#13860=ORIENTED_EDGE ( 'NONE', *, *, #7653, .F. ) ;
#13881=AXIS2_PLACEMENT_3D ( 'NONE', #17322, #3879, #10227 ) ;
#13890=VERTEX_POINT ( 'NONE', #3988 ) ;
#13902=CARTESIAN_POINT ( 'NONE',  ( -154.9999999999999716, -14.99999999999999645, 17.00000000000000000 ) ) ;
#14045=DIRECTION ( 'NONE',  ( 0.000000000000000000, 0.000000000000000000, 1.000000000000000000 ) ) ;
#14049=DIRECTION ( 'NONE',  ( 1.000000000000000000, 0.000000000000000000, -0.000000000000000000 ) ) ;
#14079=DIRECTION ( 'NONE',  ( -1.000000000000000000, 0.000000000000000000, 0.000000000000000000 ) ) ;
#14095=ORIENTED_EDGE ( 'NONE', *, *, #13531, .T. ) ;
#14126=DIRECTION ( 'NONE',  ( 0.000000000000000000, 0.000000000000000000, -1.000000000000000000 ) ) ;
#14130=ORIENTED_EDGE ( 'NONE', *, *, #13241, .T. ) ;
#14144=CARTESIAN_POINT ( 'NONE',  ( -154.9999999999999716, -14.99999999999999645, -17.00000000000000000 ) ) ;
#14156=CARTESIAN_POINT ( 'NONE',  ( -158.7998746980210001, -15.03085902363206472, 15.79999999999999893 ) ) ;
#14159=PLANE ( 'NONE',  #5876 ) ;
#14194=EDGE_CURVE ( 'NONE', #1029, #13080, #13288, .T. ) ;
#14195=CARTESIAN_POINT ( 'NONE',  ( -154.9999999999999716, -14.99999999999999645, -15.00000000000000000 ) ) ;
#14244=EDGE_LOOP ( 'NONE', ( #3436, #8288, #15928, #7096 ) ) ;
#14346=CIRCLE ( 'NONE', #18755, 3.799999999999993605 ) ;
#14369=ORIENTED_EDGE ( 'NONE', *, *, #17583, .T. ) ;
#14392=CARTESIAN_POINT ( 'NONE',  ( -155.0676494111543491, -18.79939778875158396, -15.00000000000000000 ) ) ;
#14413=EDGE_CURVE ( 'NONE', #5527, #4462, #18788, .T. ) ;
#14416=FACE_OUTER_BOUND ( 'NONE', #1571, .T. ) ;
#14438=DIRECTION ( 'NONE',  ( -2.191393683118470056E-17, -7.538405132783724027E-17, -1.000000000000000000 ) ) ;
#14468=FACE_OUTER_BOUND ( 'NONE', #16557, .T. ) ;
#14477=VERTEX_POINT ( 'NONE', #2411 ) ;
#14520=CARTESIAN_POINT ( 'NONE',  ( -155.0777214229742071, -18.79920509849242549, 15.79999999999999893 ) ) ;
#14580=VECTOR ( 'NONE', #10849, 1000.000000000000000 ) ;
#14583=ORIENTED_EDGE ( 'NONE', *, *, #5209, .F. ) ;
#14616=CIRCLE ( 'NONE', #8037, 4.000000000000031086 ) ;
#14624=CARTESIAN_POINT ( 'NONE',  ( -150.9999999999999432, -14.99999999999999645, 17.00000000000000000 ) ) ;
#14627=CYLINDRICAL_SURFACE ( 'NONE', #4980, 4.000000000000031086 ) ;
#14652=ADVANCED_FACE ( 'NONE', ( #14833 ), #14627, .T. ) ;
#14681=SHAPE_REPRESENTATION ( 'hub', ( #10359 ), #8423 ) ;
#14688=ORIENTED_EDGE ( 'NONE', *, *, #9283, .F. ) ;
#14724=DIRECTION ( 'NONE',  ( 0.9999419836444144449, 0.01077169184824096695, 0.000000000000000000 ) ) ;
#14728=LINE ( 'NONE', #14624, #5980 ) ;
#14754=ORIENTED_EDGE ( 'NONE', *, *, #6389, .F. ) ;
#14762=CARTESIAN_POINT ( 'NONE',  ( -155.0676494111543491, -18.79939778875158396, -15.79999999999999893 ) ) ;
#14770=CARTESIAN_POINT ( 'NONE',  ( -155.0676494111543491, -18.79939778875158396, -15.79999999999999893 ) ) ;
#14775=CARTESIAN_POINT ( 'NONE',  ( -154.9999999999999716, -14.99999999999999645, 15.00000000000000000 ) ) ;
#14820=LINE ( 'NONE', #16501, #15575 ) ;
#14833=FACE_OUTER_BOUND ( 'NONE', #5978, .T. ) ;
#14844=EDGE_CURVE ( 'NONE', #17411, #3719, #15878, .T. ) ;
#14850=CIRCLE ( 'NONE', #3588, 4.000000000000021316 ) ;
#14856=VERTEX_POINT ( 'NONE', #1171 ) ;
#14883=CARTESIAN_POINT ( 'NONE',  ( -154.9999999999999716, -14.99999999999999645, -15.79999999999999893 ) ) ;
#14886=ORIENTED_EDGE ( 'NONE', *, *, #8928, .T. ) ;
#14896=AXIS2_PLACEMENT_3D ( 'NONE', #16470, #16377, #17847 ) ;
#14909=EDGE_CURVE ( 'NONE', #12622, #6955, #14346, .T. ) ;
#14923=CIRCLE ( 'NONE', #516, 4.000000000000021316 ) ;
#14942=CARTESIAN_POINT ( 'NONE',  ( -154.9999999999999716, -14.99999999999999645, -15.00000000000000000 ) ) ;
#14951=ORIENTED_EDGE ( 'NONE', *, *, #8951, .T. ) ;
#14968=DIRECTION ( 'NONE',  ( -0.9999670257950099561, -0.008120795692649453515, 0.000000000000000000 ) ) ;
#15027=ADVANCED_FACE ( 'NONE', ( #4598 ), #8998, .T. ) ;
#15045=DIRECTION ( 'NONE',  ( 2.191393683118470056E-17, 7.538405132783724027E-17, 1.000000000000000000 ) ) ;
#15051=VECTOR ( 'NONE', #16167, 1000.000000000000114 ) ;
#15079=DIRECTION ( 'NONE',  ( -1.000000000000000000, 0.000000000000000000, 0.000000000000000000 ) ) ;
#15137=CARTESIAN_POINT ( 'NONE',  ( -159.0000000000000000, -14.99999999999999645, -15.79999999999999538 ) ) ;
#15243=CARTESIAN_POINT ( 'NONE',  ( -155.0818120241833640, -18.99916326157099533, 15.00000000000000000 ) ) ;
#15244=ORIENTED_EDGE ( 'NONE', *, *, #5001, .T. ) ;
#15252=AXIS2_PLACEMENT_3D ( 'NONE', #13025, #2462, #15976 ) ;
#15259=DIRECTION ( 'NONE',  ( 0.000000000000000000, 0.000000000000000000, 1.000000000000000000 ) ) ;
#15263=ORIENTED_EDGE ( 'NONE', *, *, #4008, .F. ) ;
#15337=AXIS2_PLACEMENT_3D ( 'NONE', #5115, #14126, #8340 ) ;
#15432=DIRECTION ( 'NONE',  ( 2.775466039758894710E-17, 2.253973589064049552E-19, -1.000000000000000000 ) ) ;
#15505=ORIENTED_EDGE ( 'NONE', *, *, #14909, .F. ) ;
#15508=EDGE_CURVE ( 'NONE', #4677, #8297, #2731, .T. ) ;
#15531=DIRECTION ( 'NONE',  ( 1.000000000000000000, 0.000000000000000000, 0.000000000000000000 ) ) ;
#15556=EDGE_CURVE ( 'NONE', #4857, #17995, #1551, .T. ) ;
#15563=PLANE ( 'NONE',  #13020 ) ;
#15575=VECTOR ( 'NONE', #4735, 1000.000000000000000 ) ;
#15646=DIRECTION ( 'NONE',  ( 0.03933706530295846826, -0.9992259981072103558, 7.446367396525005116E-17 ) ) ;
#15677=DIRECTION ( 'NONE',  ( 2.191393683118473446E-17, 7.538405132783725260E-17, 1.000000000000000000 ) ) ;
#15698=CIRCLE ( 'NONE', #18850, 4.000000000000031086 ) ;
#15706=CYLINDRICAL_SURFACE ( 'NONE', #353, 4.000000000000031086 ) ;
#15708=VERTEX_POINT ( 'NONE', #15243 ) ;
#15769=ORIENTED_EDGE ( 'NONE', *, *, #4601, .F. ) ;
#15777=PLANE ( 'NONE',  #4716 ) ;
#15784=CARTESIAN_POINT ( 'NONE',  ( -154.8605857259444463, -18.79744172571344762, 15.79999999999999893 ) ) ;
#15786=VERTEX_POINT ( 'NONE', #6609 ) ;
#15788=ORIENTED_EDGE ( 'NONE', *, *, #16280, .F. ) ;
#15801=ADVANCED_FACE ( 'NONE', ( #3869 ), #12887, .T. ) ;
#15809=VECTOR ( 'NONE', #1534, 1000.000000000000000 ) ;
#15831=VERTEX_POINT ( 'NONE', #2216 ) ;
#15846=CARTESIAN_POINT ( 'NONE',  ( -154.9999999999999716, -14.99999999999999645, 15.79999999999999893 ) ) ;
#15878=LINE ( 'NONE', #15784, #16244 ) ;
#15904=CIRCLE ( 'NONE', #8704, 4.000000000000031086 ) ;
#15908=DIRECTION ( 'NONE',  ( 0.9999419836444144449, 0.01077169184824096695, 0.000000000000000000 ) ) ;
#15913=DIRECTION ( 'NONE',  ( 2.191393683118470056E-17, 7.538405132783724027E-17, 1.000000000000000000 ) ) ;
#15928=ORIENTED_EDGE ( 'NONE', *, *, #15556, .T. ) ;
#15938=CARTESIAN_POINT ( 'NONE',  ( -154.8605857259444463, -18.79744172571344762, 15.79999999999999893 ) ) ;
#15948=AXIS2_PLACEMENT_3D ( 'NONE', #14144, #14045, #15531 ) ;
#15976=DIRECTION ( 'NONE',  ( 0.9999419836444144449, 0.01077169184824096695, 0.000000000000000000 ) ) ;
#16004=EDGE_LOOP ( 'NONE', ( #16820, #8590, #6048, #4940 ) ) ;
#16009=CIRCLE ( 'NONE', #979, 3.800000000000000266 ) ;
#16109=CARTESIAN_POINT ( 'NONE',  ( -154.9999999999999716, -14.99999999999999645, -15.79999999999999893 ) ) ;
#16149=DIRECTION ( 'NONE',  ( 0.000000000000000000, 0.000000000000000000, -1.000000000000000000 ) ) ;
#16167=DIRECTION ( 'NONE',  ( 0.01780247661957949992, 0.9998415233556812165, -7.576222706442768103E-17 ) ) ;
#16170=ORIENTED_EDGE ( 'NONE', *, *, #3832, .T. ) ;
#16174=DIRECTION ( 'NONE',  ( 2.191393683118473446E-17, 7.538405132783725260E-17, 1.000000000000000000 ) ) ;
#16191=DIRECTION ( 'NONE',  ( 1.000000000000000000, 0.000000000000000000, 0.000000000000000000 ) ) ;
#16244=VECTOR ( 'NONE', #2662, 1000.000000000000114 ) ;
#16259=FACE_OUTER_BOUND ( 'NONE', #16004, .T. ) ;
#16276=AXIS2_PLACEMENT_3D ( 'NONE', #10030, #9829, #14049 ) ;
#16280=EDGE_CURVE ( 'NONE', #4855, #13890, #10932, .T. ) ;
#16333=CARTESIAN_POINT ( 'NONE',  ( -155.0712099064782876, -18.99936609342274707, -15.00000000000000000 ) ) ;
#16377=DIRECTION ( 'NONE',  ( -0.000000000000000000, -0.000000000000000000, -1.000000000000000000 ) ) ;
#16383=UNCERTAINTY_MEASURE_WITH_UNIT (LENGTH_MEASURE( 1.000000000000000082E-05 ), #13001, 'distance_accuracy_value', 'NONE');
#16470=CARTESIAN_POINT ( 'NONE',  ( -154.9999999999999716, -14.99999999999999645, 17.00000000000000000 ) ) ;
#16501=CARTESIAN_POINT ( 'NONE',  ( -155.0777214229742071, -18.79920509849242549, 15.79999999999999893 ) ) ;
#16511=ORIENTED_EDGE ( 'NONE', *, *, #4590, .T. ) ;
#16551=DIRECTION ( 'NONE',  ( 0.03933706530295848214, -0.9992259981072103558, 7.446367396525006349E-17 ) ) ;
#16557=EDGE_LOOP ( 'NONE', ( #6006, #9764, #8286, #19380 ) ) ;
#16559=AXIS2_PLACEMENT_3D ( 'NONE', #13902, #398, #3438 ) ;
#16668=CIRCLE ( 'NONE', #10064, 4.000000000000031086 ) ;
#16677=DIRECTION ( 'NONE',  ( -2.191393683118470056E-17, -7.538405132783724027E-17, -1.000000000000000000 ) ) ;
#16705=ORIENTED_EDGE ( 'NONE', *, *, #2404, .F. ) ;
#16712=ORIENTED_EDGE ( 'NONE', *, *, #2404, .T. ) ;
#16758=VERTEX_POINT ( 'NONE', #17639 ) ;
#16778=ORIENTED_EDGE ( 'NONE', *, *, #9921, .T. ) ;
#16818=VECTOR ( 'NONE', #8574, 1000.000000000000000 ) ;
#16820=ORIENTED_EDGE ( 'NONE', *, *, #9283, .T. ) ;
#16935=DIRECTION ( 'NONE',  ( -0.000000000000000000, -0.000000000000000000, -1.000000000000000000 ) ) ;
#16964=UNCERTAINTY_MEASURE_WITH_UNIT (LENGTH_MEASURE( 1.000000000000000082E-05 ), #13852, 'distance_accuracy_value', 'NONE');
#16967=CARTESIAN_POINT ( 'NONE',  ( -154.9999999999999716, -14.99999999999999645, -15.79999999999999893 ) ) ;
#17038=CARTESIAN_POINT ( 'NONE',  ( -158.7997795378487353, -15.04093242902330907, -15.79999999999999893 ) ) ;
#17050=DIRECTION ( 'NONE',  ( -0.03668796685672144620, 0.9993267699245927949, 2.695122805014889898E-17 ) ) ;
#17052=LINE ( 'NONE', #8010, #17891 ) ;
#17166=VERTEX_POINT ( 'NONE', #11261 ) ;
#17218=ORIENTED_EDGE ( 'NONE', *, *, #14844, .T. ) ;
#17242=FACE_OUTER_BOUND ( 'NONE', #10656, .T. ) ;
#17322=CARTESIAN_POINT ( 'NONE',  ( -154.9999999999999716, -14.99999999999999645, 17.00000000000000000 ) ) ;
#17411=VERTEX_POINT ( 'NONE', #2760 ) ;
#17437=EDGE_CURVE ( 'NONE', #19163, #8753, #7545, .T. ) ;
#17523=DIRECTION ( 'NONE',  ( 0.000000000000000000, 0.000000000000000000, -1.000000000000000000 ) ) ;
#17525=VECTOR ( 'NONE', #16149, 1000.000000000000000 ) ;
#17536=ORIENTED_EDGE ( 'NONE', *, *, #11061, .F. ) ;
#17550=ORIENTED_EDGE ( 'NONE', *, *, #16280, .T. ) ;
#17583=EDGE_CURVE ( 'NONE', #8297, #13080, #12550, .T. ) ;
#17639=CARTESIAN_POINT ( 'NONE',  ( -150.9999999999999432, -14.99999999999999645, 17.00000000000000000 ) ) ;
#17657=ORIENTED_EDGE ( 'NONE', *, *, #13363, .T. ) ;
#17703=CIRCLE ( 'NONE', #10489, 3.800000000000000266 ) ;
#17847=DIRECTION ( 'NONE',  ( -1.000000000000000000, 0.000000000000000000, 0.000000000000000000 ) ) ;
#17891=VECTOR ( 'NONE', #3810, 1000.000000000000000 ) ;
#17995=VERTEX_POINT ( 'NONE', #19364 ) ;
#17996=LINE ( 'NONE', #3190, #3058 ) ;
#18009=ORIENTED_EDGE ( 'NONE', *, *, #15556, .F. ) ;
#18010=ORIENTED_EDGE ( 'NONE', *, *, #3832, .F. ) ;
#18020=CYLINDRICAL_SURFACE ( 'NONE', #1932, 3.800000000000000266 ) ;
#18046=ORIENTED_EDGE ( 'NONE', *, *, #10467, .T. ) ;
#18052=VECTOR ( 'NONE', #2253, 1000.000000000000000 ) ;
#18104=CIRCLE ( 'NONE', #15252, 3.799999999999993605 ) ;
#18134=VECTOR ( 'NONE', #5471, 1000.000000000000000 ) ;
#18154=STYLED_ITEM ( 'NONE', ( #11519 ), #1480 ) ;
#18191=AXIS2_PLACEMENT_3D ( 'NONE', #14775, #2746, #15079 ) ;
#18195=AXIS2_PLACEMENT_3D ( 'NONE', #7864, #223, #12079 ) ;
#18196=DIRECTION ( 'NONE',  ( 2.191393683118470056E-17, 7.538405132783724027E-17, 1.000000000000000000 ) ) ;
#18201=CARTESIAN_POINT ( 'NONE',  ( -155.0777214229742071, -18.79920509849242549, 15.79999999999999893 ) ) ;
#18210=ORIENTED_EDGE ( 'NONE', *, *, #6811, .T. ) ;
#18258=ORIENTED_EDGE ( 'NONE', *, *, #13241, .F. ) ;
#18263=DIRECTION ( 'NONE',  ( 0.01780247661957949992, 0.9998415233556812165, -7.576222706442768103E-17 ) ) ;
#18287=CARTESIAN_POINT ( 'NONE',  ( -154.9999999999999716, -14.99999999999999645, -15.00000000000000000 ) ) ;
#18306=ORIENTED_EDGE ( 'NONE', *, *, #12522, .F. ) ;
#18324=ADVANCED_FACE ( 'NONE', ( #14468 ), #8493, .T. ) ;
#18329=CIRCLE ( 'NONE', #158, 3.799999999999993605 ) ;
#18346=DIRECTION ( 'NONE',  ( 0.9999419836444144449, 0.01077169184824096695, 0.000000000000000000 ) ) ;
#18349=CYLINDRICAL_SURFACE ( 'NONE', #7837, 3.800000000000000266 ) ;
#18455=ORIENTED_EDGE ( 'NONE', *, *, #3244, .F. ) ;
#18515=LINE ( 'NONE', #3313, #994 ) ;
#18624=CYLINDRICAL_SURFACE ( 'NONE', #9564, 4.000000000000031086 ) ;
#18634=CARTESIAN_POINT ( 'NONE',  ( -154.9999999999999716, -14.99999999999999645, 15.79999999999999893 ) ) ;
#18642=ADVANCED_FACE ( 'NONE', ( #2911 ), #8872, .T. ) ;
#18651=CIRCLE ( 'NONE', #4546, 3.799999999999993605 ) ;
#18718=LINE ( 'NONE', #9570, #14580 ) ;
#18755=AXIS2_PLACEMENT_3D ( 'NONE', #14195, #9788, #778 ) ;
#18788=CIRCLE ( 'NONE', #15948, 4.000000000000031086 ) ;
#18850=AXIS2_PLACEMENT_3D ( 'NONE', #11616, #13284, #19204 ) ;
#18869=FACE_OUTER_BOUND ( 'NONE', #12978, .T. ) ;
#18870=ORIENTED_EDGE ( 'NONE', *, *, #8928, .F. ) ;
#18875=CARTESIAN_POINT ( 'NONE',  ( -159.0000000000000000, -14.99999999999999645, 17.00000000000000000 ) ) ;
#18895=DIRECTION ( 'NONE',  ( 0.000000000000000000, 0.000000000000000000, 1.000000000000000000 ) ) ;
#18934=CIRCLE ( 'NONE', #7010, 3.799999999999993605 ) ;
#19003=ORIENTED_EDGE ( 'NONE', *, *, #12790, .T. ) ;
#19007=( NAMED_UNIT ( * ) PLANE_ANGLE_UNIT ( ) SI_UNIT ( $, .RADIAN. ) );
#19015=EDGE_CURVE ( 'NONE', #19163, #4462, #14728, .T. ) ;
#19069=DIRECTION ( 'NONE',  ( 0.000000000000000000, -1.000000000000000000, 0.000000000000000000 ) ) ;
#19107=( NAMED_UNIT ( * ) PLANE_ANGLE_UNIT ( ) SI_UNIT ( $, .RADIAN. ) );
#19137=ORIENTED_EDGE ( 'NONE', *, *, #5209, .T. ) ;
#19163=VERTEX_POINT ( 'NONE', #1699 ) ;
#19204=DIRECTION ( 'NONE',  ( -1.000000000000000000, 0.000000000000000000, 0.000000000000000000 ) ) ;
#19210=ORIENTED_EDGE ( 'NONE', *, *, #6389, .T. ) ;
#19214=ORIENTED_EDGE ( 'NONE', *, *, #11972, .F. ) ;
#19234=ORIENTED_EDGE ( 'NONE', *, *, #14413, .T. ) ;
#19264=ADVANCED_FACE ( 'NONE', ( #6108 ), #13742, .T. ) ;
#19315=CARTESIAN_POINT ( 'NONE',  ( -154.9999999999999716, -14.99999999999999645, 15.00000000000000000 ) ) ;
#19364=CARTESIAN_POINT ( 'NONE',  ( -155.0777214229742071, -18.79920509849242549, 15.00000000000000000 ) ) ;
#19380=ORIENTED_EDGE ( 'NONE', *, *, #3081, .F. ) ;
#19405=CARTESIAN_POINT ( 'NONE',  ( -151.2001253019789431, -14.96914097636792818, 15.79999999999999893 ) ) ;
#19476=COLOUR_RGB('Off White',0.89,0.88,0.83);
#19477=FILL_AREA_STYLE_COLOUR('',#19476);
#19478=FILL_AREA_STYLE('',(#19477));
#19479=SURFACE_STYLE_FILL_AREA(#19478);
#19480=SURFACE_SIDE_STYLE('',(#19479));
#19481=SURFACE_STYLE_USAGE(.BOTH.,#19480);
#19482=PRESENTATION_STYLE_ASSIGNMENT((#19481));
ENDSEC;
END-ISO-10303-21;
